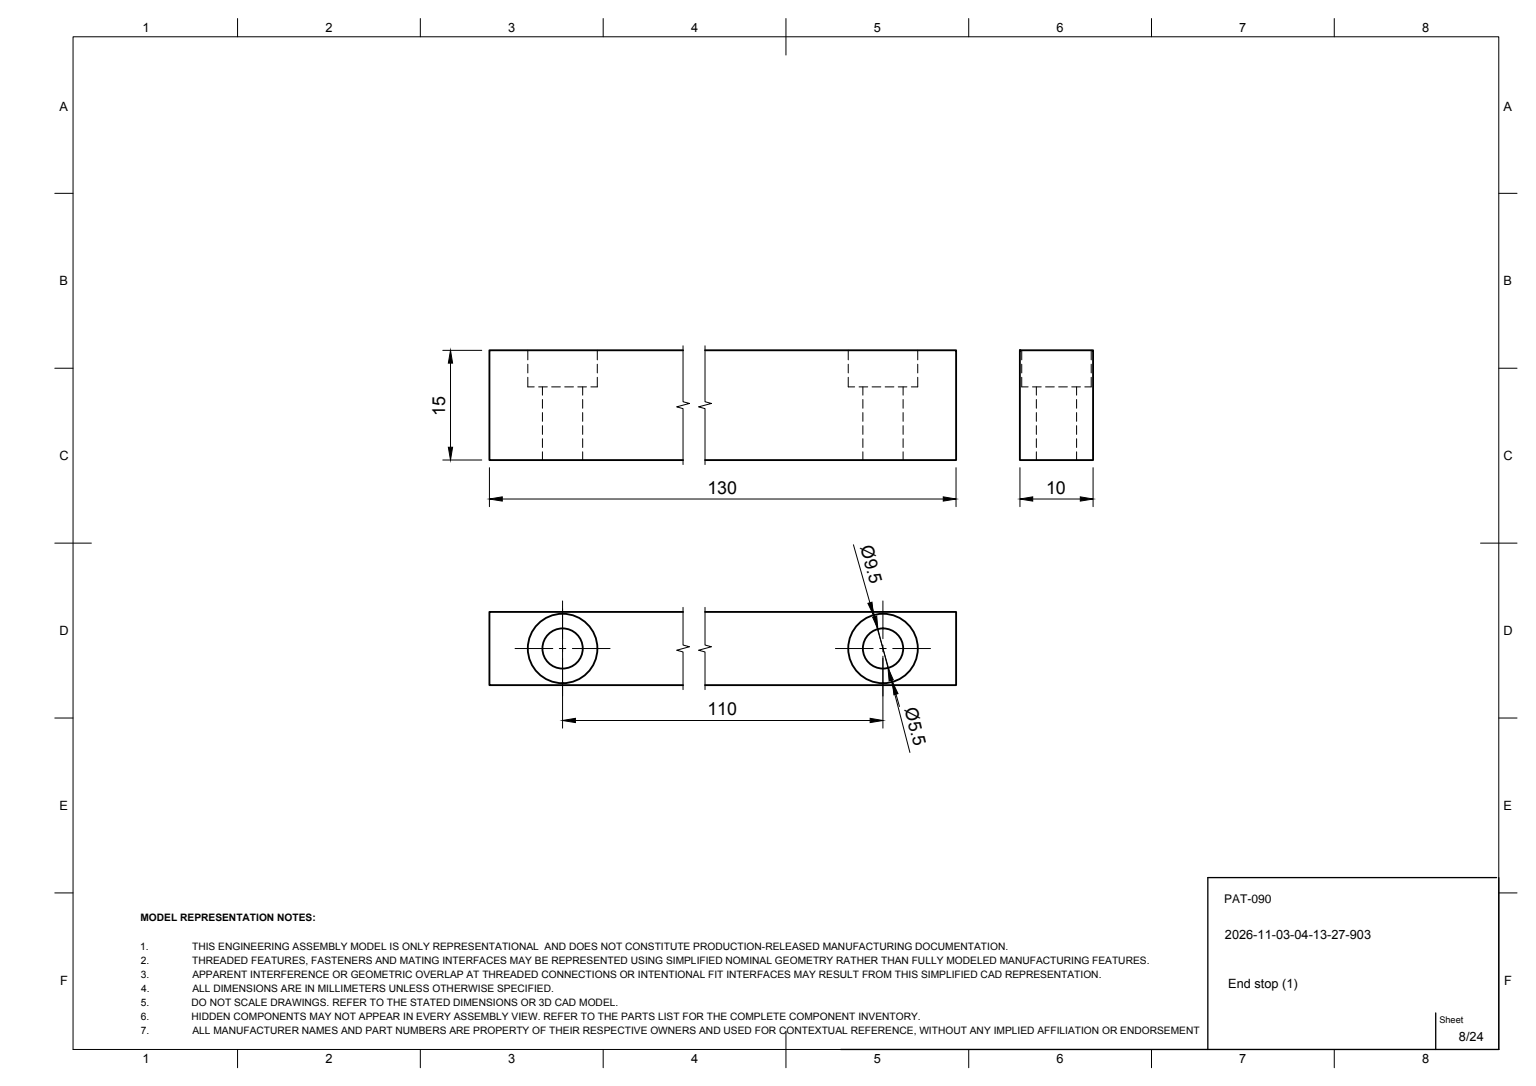
ISO-10303-21;
HEADER;
/* Generated by software containing ST-Developer
 * from STEP Tools, Inc. (www.steptools.com) 
 */

FILE_DESCRIPTION(
/* description */ ('Round-Shaft Linear Stage with Ball Bushings'),
/* implementation_level */ '2;1');

FILE_NAME(
/* name */ 'End stop (1).step',
/* time_stamp */ '2026-10-27T10:47:55-07:00',
/* author */ (''),
/* organization */ (''),
/* preprocessor_version */ 'ST-DEVELOPER v20.2',
/* originating_system */ 'Autodesk Translation Framework v15.17.0.0',
/* authorisation */ '');

FILE_SCHEMA (('AUTOMOTIVE_DESIGN { 1 0 10303 214 3 1 1 }'));
ENDSEC;

DATA;
#10=MECHANICAL_DESIGN_GEOMETRIC_PRESENTATION_REPRESENTATION('',(#305),#7835);
#263=SHAPE_REPRESENTATION_RELATIONSHIP('SRR','None',#7951,#284);
#284=ADVANCED_BREP_SHAPE_REPRESENTATION('',(#326),#7815);
#305=STYLED_ITEM('',(#8137),#326);
#326=MANIFOLD_SOLID_BREP('Body1',#4395);
#370=FACE_BOUND('',#941,.T.);
#371=FACE_BOUND('',#944,.T.);
#372=FACE_BOUND('',#952,.T.);
#373=FACE_BOUND('',#953,.T.);
#374=FACE_BOUND('',#955,.T.);
#375=FACE_BOUND('',#956,.T.);
#479=PLANE('',#4726);
#480=PLANE('',#4731);
#481=PLANE('',#4737);
#482=PLANE('',#4738);
#483=PLANE('',#4739);
#484=PLANE('',#4740);
#485=PLANE('',#4741);
#486=PLANE('',#4742);
#652=FACE_OUTER_BOUND('',#939,.T.);
#653=FACE_OUTER_BOUND('',#940,.T.);
#654=FACE_OUTER_BOUND('',#942,.T.);
#655=FACE_OUTER_BOUND('',#943,.T.);
#656=FACE_OUTER_BOUND('',#945,.T.);
#657=FACE_OUTER_BOUND('',#946,.T.);
#658=FACE_OUTER_BOUND('',#947,.T.);
#659=FACE_OUTER_BOUND('',#948,.T.);
#660=FACE_OUTER_BOUND('',#949,.T.);
#661=FACE_OUTER_BOUND('',#950,.T.);
#662=FACE_OUTER_BOUND('',#951,.T.);
#663=FACE_OUTER_BOUND('',#954,.T.);
#939=EDGE_LOOP('',(#3162,#3163,#3164,#3165));
#940=EDGE_LOOP('',(#3166));
#941=EDGE_LOOP('',(#3167));
#942=EDGE_LOOP('',(#3168,#3169,#3170,#3171));
#943=EDGE_LOOP('',(#3172));
#944=EDGE_LOOP('',(#3173));
#945=EDGE_LOOP('',(#3174,#3175,#3176,#3177));
#946=EDGE_LOOP('',(#3178,#3179,#3180,#3181));
#947=EDGE_LOOP('',(#3182,#3183,#3184,#3185));
#948=EDGE_LOOP('',(#3186,#3187,#3188,#3189));
#949=EDGE_LOOP('',(#3190,#3191,#3192,#3193));
#950=EDGE_LOOP('',(#3194,#3195,#3196,#3197));
#951=EDGE_LOOP('',(#3198,#3199,#3200,#3201));
#952=EDGE_LOOP('',(#3202));
#953=EDGE_LOOP('',(#3203));
#954=EDGE_LOOP('',(#3204,#3205,#3206,#3207));
#955=EDGE_LOOP('',(#3208));
#956=EDGE_LOOP('',(#3209));
#1301=LINE('',#6756,#1641);
#1302=LINE('',#6765,#1642);
#1303=LINE('',#6773,#1643);
#1304=LINE('',#6777,#1644);
#1305=LINE('',#6781,#1645);
#1306=LINE('',#6783,#1646);
#1307=LINE('',#6785,#1647);
#1308=LINE('',#6786,#1648);
#1309=LINE('',#6789,#1649);
#1310=LINE('',#6791,#1650);
#1311=LINE('',#6792,#1651);
#1312=LINE('',#6795,#1652);
#1313=LINE('',#6797,#1653);
#1314=LINE('',#6798,#1654);
#1315=LINE('',#6800,#1655);
#1316=LINE('',#6801,#1656);
#1641=VECTOR('',#5380,0.475000000000001);
#1642=VECTOR('',#5391,0.475000000000001);
#1643=VECTOR('',#5402,0.274999999999999);
#1644=VECTOR('',#5407,0.274999999999999);
#1645=VECTOR('',#5410,1.);
#1646=VECTOR('',#5411,1.);
#1647=VECTOR('',#5412,1.);
#1648=VECTOR('',#5413,1.);
#1649=VECTOR('',#5416,1.);
#1650=VECTOR('',#5417,1.);
#1651=VECTOR('',#5418,1.);
#1652=VECTOR('',#5421,1.);
#1653=VECTOR('',#5422,1.);
#1654=VECTOR('',#5423,1.);
#1655=VECTOR('',#5426,1.);
#1656=VECTOR('',#5427,1.);
#1961=CIRCLE('',#4724,0.475000000000001);
#1962=CIRCLE('',#4725,0.475000000000001);
#1963=CIRCLE('',#4727,0.274999999999999);
#1964=CIRCLE('',#4729,0.475000000000001);
#1965=CIRCLE('',#4730,0.475000000000001);
#1966=CIRCLE('',#4732,0.274999999999999);
#1967=CIRCLE('',#4734,0.274999999999999);
#1968=CIRCLE('',#4736,0.274999999999999);
#2174=VERTEX_POINT('',#6753);
#2175=VERTEX_POINT('',#6755);
#2176=VERTEX_POINT('',#6759);
#2177=VERTEX_POINT('',#6762);
#2178=VERTEX_POINT('',#6764);
#2179=VERTEX_POINT('',#6768);
#2180=VERTEX_POINT('',#6771);
#2181=VERTEX_POINT('',#6775);
#2182=VERTEX_POINT('',#6779);
#2183=VERTEX_POINT('',#6780);
#2184=VERTEX_POINT('',#6782);
#2185=VERTEX_POINT('',#6784);
#2186=VERTEX_POINT('',#6788);
#2187=VERTEX_POINT('',#6790);
#2188=VERTEX_POINT('',#6794);
#2189=VERTEX_POINT('',#6796);
#2549=EDGE_CURVE('',#2174,#2174,#1961,.T.);
#2550=EDGE_CURVE('',#2174,#2175,#1301,.T.);
#2551=EDGE_CURVE('',#2175,#2175,#1962,.T.);
#2552=EDGE_CURVE('',#2176,#2176,#1963,.T.);
#2553=EDGE_CURVE('',#2177,#2177,#1964,.T.);
#2554=EDGE_CURVE('',#2177,#2178,#1302,.T.);
#2555=EDGE_CURVE('',#2178,#2178,#1965,.T.);
#2556=EDGE_CURVE('',#2179,#2179,#1966,.T.);
#2557=EDGE_CURVE('',#2180,#2180,#1967,.T.);
#2558=EDGE_CURVE('',#2180,#2176,#1303,.T.);
#2559=EDGE_CURVE('',#2181,#2181,#1968,.T.);
#2560=EDGE_CURVE('',#2181,#2179,#1304,.T.);
#2561=EDGE_CURVE('',#2182,#2183,#1305,.T.);
#2562=EDGE_CURVE('',#2183,#2184,#1306,.T.);
#2563=EDGE_CURVE('',#2185,#2184,#1307,.T.);
#2564=EDGE_CURVE('',#2182,#2185,#1308,.T.);
#2565=EDGE_CURVE('',#2186,#2182,#1309,.T.);
#2566=EDGE_CURVE('',#2187,#2185,#1310,.T.);
#2567=EDGE_CURVE('',#2186,#2187,#1311,.T.);
#2568=EDGE_CURVE('',#2188,#2186,#1312,.T.);
#2569=EDGE_CURVE('',#2189,#2187,#1313,.T.);
#2570=EDGE_CURVE('',#2188,#2189,#1314,.T.);
#2571=EDGE_CURVE('',#2183,#2188,#1315,.T.);
#2572=EDGE_CURVE('',#2184,#2189,#1316,.T.);
#3162=ORIENTED_EDGE('',*,*,#2549,.F.);
#3163=ORIENTED_EDGE('',*,*,#2550,.T.);
#3164=ORIENTED_EDGE('',*,*,#2551,.F.);
#3165=ORIENTED_EDGE('',*,*,#2550,.F.);
#3166=ORIENTED_EDGE('',*,*,#2549,.T.);
#3167=ORIENTED_EDGE('',*,*,#2552,.F.);
#3168=ORIENTED_EDGE('',*,*,#2553,.F.);
#3169=ORIENTED_EDGE('',*,*,#2554,.T.);
#3170=ORIENTED_EDGE('',*,*,#2555,.F.);
#3171=ORIENTED_EDGE('',*,*,#2554,.F.);
#3172=ORIENTED_EDGE('',*,*,#2553,.T.);
#3173=ORIENTED_EDGE('',*,*,#2556,.F.);
#3174=ORIENTED_EDGE('',*,*,#2557,.F.);
#3175=ORIENTED_EDGE('',*,*,#2558,.T.);
#3176=ORIENTED_EDGE('',*,*,#2552,.T.);
#3177=ORIENTED_EDGE('',*,*,#2558,.F.);
#3178=ORIENTED_EDGE('',*,*,#2559,.F.);
#3179=ORIENTED_EDGE('',*,*,#2560,.T.);
#3180=ORIENTED_EDGE('',*,*,#2556,.T.);
#3181=ORIENTED_EDGE('',*,*,#2560,.F.);
#3182=ORIENTED_EDGE('',*,*,#2561,.T.);
#3183=ORIENTED_EDGE('',*,*,#2562,.T.);
#3184=ORIENTED_EDGE('',*,*,#2563,.F.);
#3185=ORIENTED_EDGE('',*,*,#2564,.F.);
#3186=ORIENTED_EDGE('',*,*,#2565,.T.);
#3187=ORIENTED_EDGE('',*,*,#2564,.T.);
#3188=ORIENTED_EDGE('',*,*,#2566,.F.);
#3189=ORIENTED_EDGE('',*,*,#2567,.F.);
#3190=ORIENTED_EDGE('',*,*,#2568,.T.);
#3191=ORIENTED_EDGE('',*,*,#2567,.T.);
#3192=ORIENTED_EDGE('',*,*,#2569,.F.);
#3193=ORIENTED_EDGE('',*,*,#2570,.F.);
#3194=ORIENTED_EDGE('',*,*,#2571,.T.);
#3195=ORIENTED_EDGE('',*,*,#2570,.T.);
#3196=ORIENTED_EDGE('',*,*,#2572,.F.);
#3197=ORIENTED_EDGE('',*,*,#2562,.F.);
#3198=ORIENTED_EDGE('',*,*,#2572,.T.);
#3199=ORIENTED_EDGE('',*,*,#2569,.T.);
#3200=ORIENTED_EDGE('',*,*,#2566,.T.);
#3201=ORIENTED_EDGE('',*,*,#2563,.T.);
#3202=ORIENTED_EDGE('',*,*,#2551,.T.);
#3203=ORIENTED_EDGE('',*,*,#2555,.T.);
#3204=ORIENTED_EDGE('',*,*,#2571,.F.);
#3205=ORIENTED_EDGE('',*,*,#2561,.F.);
#3206=ORIENTED_EDGE('',*,*,#2565,.F.);
#3207=ORIENTED_EDGE('',*,*,#2568,.F.);
#3208=ORIENTED_EDGE('',*,*,#2557,.T.);
#3209=ORIENTED_EDGE('',*,*,#2559,.T.);
#4068=CYLINDRICAL_SURFACE('',#4723,0.475000000000001);
#4069=CYLINDRICAL_SURFACE('',#4728,0.475000000000001);
#4070=CYLINDRICAL_SURFACE('',#4733,0.274999999999999);
#4071=CYLINDRICAL_SURFACE('',#4735,0.274999999999999);
#4171=ADVANCED_FACE('',(#652),#4068,.F.);
#4172=ADVANCED_FACE('',(#653,#370),#479,.T.);
#4173=ADVANCED_FACE('',(#654),#4069,.F.);
#4174=ADVANCED_FACE('',(#655,#371),#480,.T.);
#4175=ADVANCED_FACE('',(#656),#4070,.F.);
#4176=ADVANCED_FACE('',(#657),#4071,.F.);
#4177=ADVANCED_FACE('',(#658),#481,.T.);
#4178=ADVANCED_FACE('',(#659),#482,.T.);
#4179=ADVANCED_FACE('',(#660),#483,.T.);
#4180=ADVANCED_FACE('',(#661),#484,.T.);
#4181=ADVANCED_FACE('',(#662,#372,#373),#485,.T.);
#4182=ADVANCED_FACE('',(#663,#374,#375),#486,.F.);
#4395=CLOSED_SHELL('',(#4171,#4172,#4173,#4174,#4175,#4176,#4177,#4178,
#4179,#4180,#4181,#4182));
#4722=AXIS2_PLACEMENT_3D('',#6751,#5374,#5375);
#4723=AXIS2_PLACEMENT_3D('',#6752,#5376,#5377);
#4724=AXIS2_PLACEMENT_3D('',#6754,#5378,#5379);
#4725=AXIS2_PLACEMENT_3D('',#6757,#5381,#5382);
#4726=AXIS2_PLACEMENT_3D('',#6758,#5383,#5384);
#4727=AXIS2_PLACEMENT_3D('',#6760,#5385,#5386);
#4728=AXIS2_PLACEMENT_3D('',#6761,#5387,#5388);
#4729=AXIS2_PLACEMENT_3D('',#6763,#5389,#5390);
#4730=AXIS2_PLACEMENT_3D('',#6766,#5392,#5393);
#4731=AXIS2_PLACEMENT_3D('',#6767,#5394,#5395);
#4732=AXIS2_PLACEMENT_3D('',#6769,#5396,#5397);
#4733=AXIS2_PLACEMENT_3D('',#6770,#5398,#5399);
#4734=AXIS2_PLACEMENT_3D('',#6772,#5400,#5401);
#4735=AXIS2_PLACEMENT_3D('',#6774,#5403,#5404);
#4736=AXIS2_PLACEMENT_3D('',#6776,#5405,#5406);
#4737=AXIS2_PLACEMENT_3D('',#6778,#5408,#5409);
#4738=AXIS2_PLACEMENT_3D('',#6787,#5414,#5415);
#4739=AXIS2_PLACEMENT_3D('',#6793,#5419,#5420);
#4740=AXIS2_PLACEMENT_3D('',#6799,#5424,#5425);
#4741=AXIS2_PLACEMENT_3D('',#6802,#5428,#5429);
#4742=AXIS2_PLACEMENT_3D('',#6803,#5430,#5431);
#5374=DIRECTION('axis',(0.,0.,1.));
#5375=DIRECTION('refdir',(1.,0.,0.));
#5376=DIRECTION('center_axis',(0.,0.,1.));
#5377=DIRECTION('ref_axis',(1.,0.,0.));
#5378=DIRECTION('center_axis',(0.,0.,1.));
#5379=DIRECTION('ref_axis',(1.,0.,0.));
#5380=DIRECTION('',(0.,0.,1.));
#5381=DIRECTION('center_axis',(0.,0.,-1.));
#5382=DIRECTION('ref_axis',(1.,0.,0.));
#5383=DIRECTION('center_axis',(0.,0.,1.));
#5384=DIRECTION('ref_axis',(1.,0.,0.));
#5385=DIRECTION('center_axis',(0.,0.,1.));
#5386=DIRECTION('ref_axis',(1.,0.,0.));
#5387=DIRECTION('center_axis',(0.,0.,1.));
#5388=DIRECTION('ref_axis',(1.,0.,0.));
#5389=DIRECTION('center_axis',(0.,0.,1.));
#5390=DIRECTION('ref_axis',(1.,0.,0.));
#5391=DIRECTION('',(0.,0.,1.));
#5392=DIRECTION('center_axis',(0.,0.,-1.));
#5393=DIRECTION('ref_axis',(1.,0.,0.));
#5394=DIRECTION('center_axis',(0.,0.,1.));
#5395=DIRECTION('ref_axis',(1.,0.,0.));
#5396=DIRECTION('center_axis',(0.,0.,1.));
#5397=DIRECTION('ref_axis',(1.,0.,0.));
#5398=DIRECTION('center_axis',(0.,0.,1.));
#5399=DIRECTION('ref_axis',(1.,0.,0.));
#5400=DIRECTION('center_axis',(0.,0.,1.));
#5401=DIRECTION('ref_axis',(1.,0.,0.));
#5402=DIRECTION('',(0.,0.,1.));
#5403=DIRECTION('center_axis',(0.,0.,1.));
#5404=DIRECTION('ref_axis',(1.,0.,0.));
#5405=DIRECTION('center_axis',(0.,0.,1.));
#5406=DIRECTION('ref_axis',(1.,0.,0.));
#5407=DIRECTION('',(0.,0.,1.));
#5408=DIRECTION('center_axis',(0.,1.,0.));
#5409=DIRECTION('ref_axis',(-1.,0.,0.));
#5410=DIRECTION('',(-1.,0.,0.));
#5411=DIRECTION('',(0.,0.,1.));
#5412=DIRECTION('',(-1.,0.,0.));
#5413=DIRECTION('',(0.,0.,1.));
#5414=DIRECTION('center_axis',(1.,0.,0.));
#5415=DIRECTION('ref_axis',(0.,1.,0.));
#5416=DIRECTION('',(0.,1.,0.));
#5417=DIRECTION('',(0.,1.,0.));
#5418=DIRECTION('',(0.,0.,1.));
#5419=DIRECTION('center_axis',(0.,-1.,0.));
#5420=DIRECTION('ref_axis',(1.,0.,0.));
#5421=DIRECTION('',(1.,0.,0.));
#5422=DIRECTION('',(1.,0.,0.));
#5423=DIRECTION('',(0.,0.,1.));
#5424=DIRECTION('center_axis',(-1.,0.,0.));
#5425=DIRECTION('ref_axis',(0.,-1.,0.));
#5426=DIRECTION('',(0.,-1.,0.));
#5427=DIRECTION('',(0.,-1.,0.));
#5428=DIRECTION('center_axis',(0.,0.,1.));
#5429=DIRECTION('ref_axis',(1.,0.,0.));
#5430=DIRECTION('center_axis',(0.,0.,1.));
#5431=DIRECTION('ref_axis',(1.,0.,0.));
#6751=CARTESIAN_POINT('',(0.,0.,0.));
#6752=CARTESIAN_POINT('Origin',(26.5,-5.5,2.));
#6753=CARTESIAN_POINT('',(26.025,-5.5,2.));
#6754=CARTESIAN_POINT('Origin',(26.5,-5.5,2.));
#6755=CARTESIAN_POINT('',(26.025,-5.5,2.5));
#6756=CARTESIAN_POINT('',(26.025,-5.5,2.));
#6757=CARTESIAN_POINT('Origin',(26.5,-5.5,2.5));
#6758=CARTESIAN_POINT('Origin',(26.5,-5.5,2.));
#6759=CARTESIAN_POINT('',(26.225,-5.5,2.));
#6760=CARTESIAN_POINT('Origin',(26.5,-5.5,2.));
#6761=CARTESIAN_POINT('Origin',(26.5,5.5,2.));
#6762=CARTESIAN_POINT('',(26.025,5.5,2.));
#6763=CARTESIAN_POINT('Origin',(26.5,5.5,2.));
#6764=CARTESIAN_POINT('',(26.025,5.5,2.5));
#6765=CARTESIAN_POINT('',(26.025,5.5,2.));
#6766=CARTESIAN_POINT('Origin',(26.5,5.5,2.5));
#6767=CARTESIAN_POINT('Origin',(26.5,5.5,2.));
#6768=CARTESIAN_POINT('',(26.225,5.5,2.));
#6769=CARTESIAN_POINT('Origin',(26.5,5.5,2.));
#6770=CARTESIAN_POINT('Origin',(26.5,-5.5,0.9));
#6771=CARTESIAN_POINT('',(26.225,-5.5,1.));
#6772=CARTESIAN_POINT('Origin',(26.5,-5.5,1.));
#6773=CARTESIAN_POINT('',(26.225,-5.5,0.9));
#6774=CARTESIAN_POINT('Origin',(26.5,5.5,0.9));
#6775=CARTESIAN_POINT('',(26.225,5.5,1.));
#6776=CARTESIAN_POINT('Origin',(26.5,5.5,1.));
#6777=CARTESIAN_POINT('',(26.225,5.5,0.9));
#6778=CARTESIAN_POINT('Origin',(27.,6.5,1.));
#6779=CARTESIAN_POINT('',(27.,6.5,1.));
#6780=CARTESIAN_POINT('',(26.,6.5,1.));
#6781=CARTESIAN_POINT('',(27.,6.5,1.));
#6782=CARTESIAN_POINT('',(26.,6.5,2.5));
#6783=CARTESIAN_POINT('',(26.,6.5,1.));
#6784=CARTESIAN_POINT('',(27.,6.5,2.5));
#6785=CARTESIAN_POINT('',(27.,6.5,2.5));
#6786=CARTESIAN_POINT('',(27.,6.5,1.));
#6787=CARTESIAN_POINT('Origin',(27.,-6.5,1.));
#6788=CARTESIAN_POINT('',(27.,-6.5,1.));
#6789=CARTESIAN_POINT('',(27.,-6.5,1.));
#6790=CARTESIAN_POINT('',(27.,-6.5,2.5));
#6791=CARTESIAN_POINT('',(27.,-6.5,2.5));
#6792=CARTESIAN_POINT('',(27.,-6.5,1.));
#6793=CARTESIAN_POINT('Origin',(26.,-6.5,1.));
#6794=CARTESIAN_POINT('',(26.,-6.5,1.));
#6795=CARTESIAN_POINT('',(26.,-6.5,1.));
#6796=CARTESIAN_POINT('',(26.,-6.5,2.5));
#6797=CARTESIAN_POINT('',(26.,-6.5,2.5));
#6798=CARTESIAN_POINT('',(26.,-6.5,1.));
#6799=CARTESIAN_POINT('Origin',(26.,6.5,1.));
#6800=CARTESIAN_POINT('',(26.,6.5,1.));
#6801=CARTESIAN_POINT('',(26.,6.5,2.5));
#6802=CARTESIAN_POINT('Origin',(26.5,0.,2.5));
#6803=CARTESIAN_POINT('Origin',(26.5,0.,1.));
#7789=UNCERTAINTY_MEASURE_WITH_UNIT(LENGTH_MEASURE(0.001),#7836,
'DISTANCE_ACCURACY_VALUE',
'Maximum model space distance between geometric entities at asserted c
onnectivities');
#7809=UNCERTAINTY_MEASURE_WITH_UNIT(LENGTH_MEASURE(0.001),#7836,
'DISTANCE_ACCURACY_VALUE',
'Maximum model space distance between geometric entities at asserted c
onnectivities');
#7815=(
GEOMETRIC_REPRESENTATION_CONTEXT(3)
GLOBAL_UNCERTAINTY_ASSIGNED_CONTEXT((#7789))
GLOBAL_UNIT_ASSIGNED_CONTEXT((#7836,#7838,#7839))
REPRESENTATION_CONTEXT('','3D')
);
#7835=(
GEOMETRIC_REPRESENTATION_CONTEXT(3)
GLOBAL_UNCERTAINTY_ASSIGNED_CONTEXT((#7809))
GLOBAL_UNIT_ASSIGNED_CONTEXT((#7836,#7838,#7839))
REPRESENTATION_CONTEXT('','3D')
);
#7836=(
LENGTH_UNIT()
NAMED_UNIT(*)
SI_UNIT(.CENTI.,.METRE.)
);
#7838=(
NAMED_UNIT(*)
PLANE_ANGLE_UNIT()
SI_UNIT($,.RADIAN.)
);
#7839=(
NAMED_UNIT(*)
SI_UNIT($,.STERADIAN.)
SOLID_ANGLE_UNIT()
);
#7845=SHAPE_DEFINITION_REPRESENTATION(#7870,#7951);
#7870=PRODUCT_DEFINITION_SHAPE('',$,#7977);
#7951=SHAPE_REPRESENTATION('',(#4722),#7815);
#7971=PRODUCT_DEFINITION_CONTEXT('part definition',#8048,'design');
#7977=PRODUCT_DEFINITION('End stop (1)','End stop (1)',#8002,#7971);
#8002=PRODUCT_DEFINITION_FORMATION('',$,#8055);
#8048=APPLICATION_CONTEXT(
'Core Data for Automotive Mechanical Design Process');
#8049=PRODUCT_CONTEXT('part definition',#8048,'mechanical');
#8055=PRODUCT('End stop (1)','End stop (1)','End stop (1)',(#8049));
#8131=COLOUR_RGB('Sky Blue',0.24,0.69,0.87);
#8132=FILL_AREA_STYLE_COLOUR('',#8131);
#8133=FILL_AREA_STYLE('',(#8132));
#8134=SURFACE_STYLE_FILL_AREA(#8133);
#8135=SURFACE_SIDE_STYLE('',(#8134));
#8136=SURFACE_STYLE_USAGE(.BOTH.,#8135);
#8137=PRESENTATION_STYLE_ASSIGNMENT((#8136));
ENDSEC;
END-ISO-10303-21;
